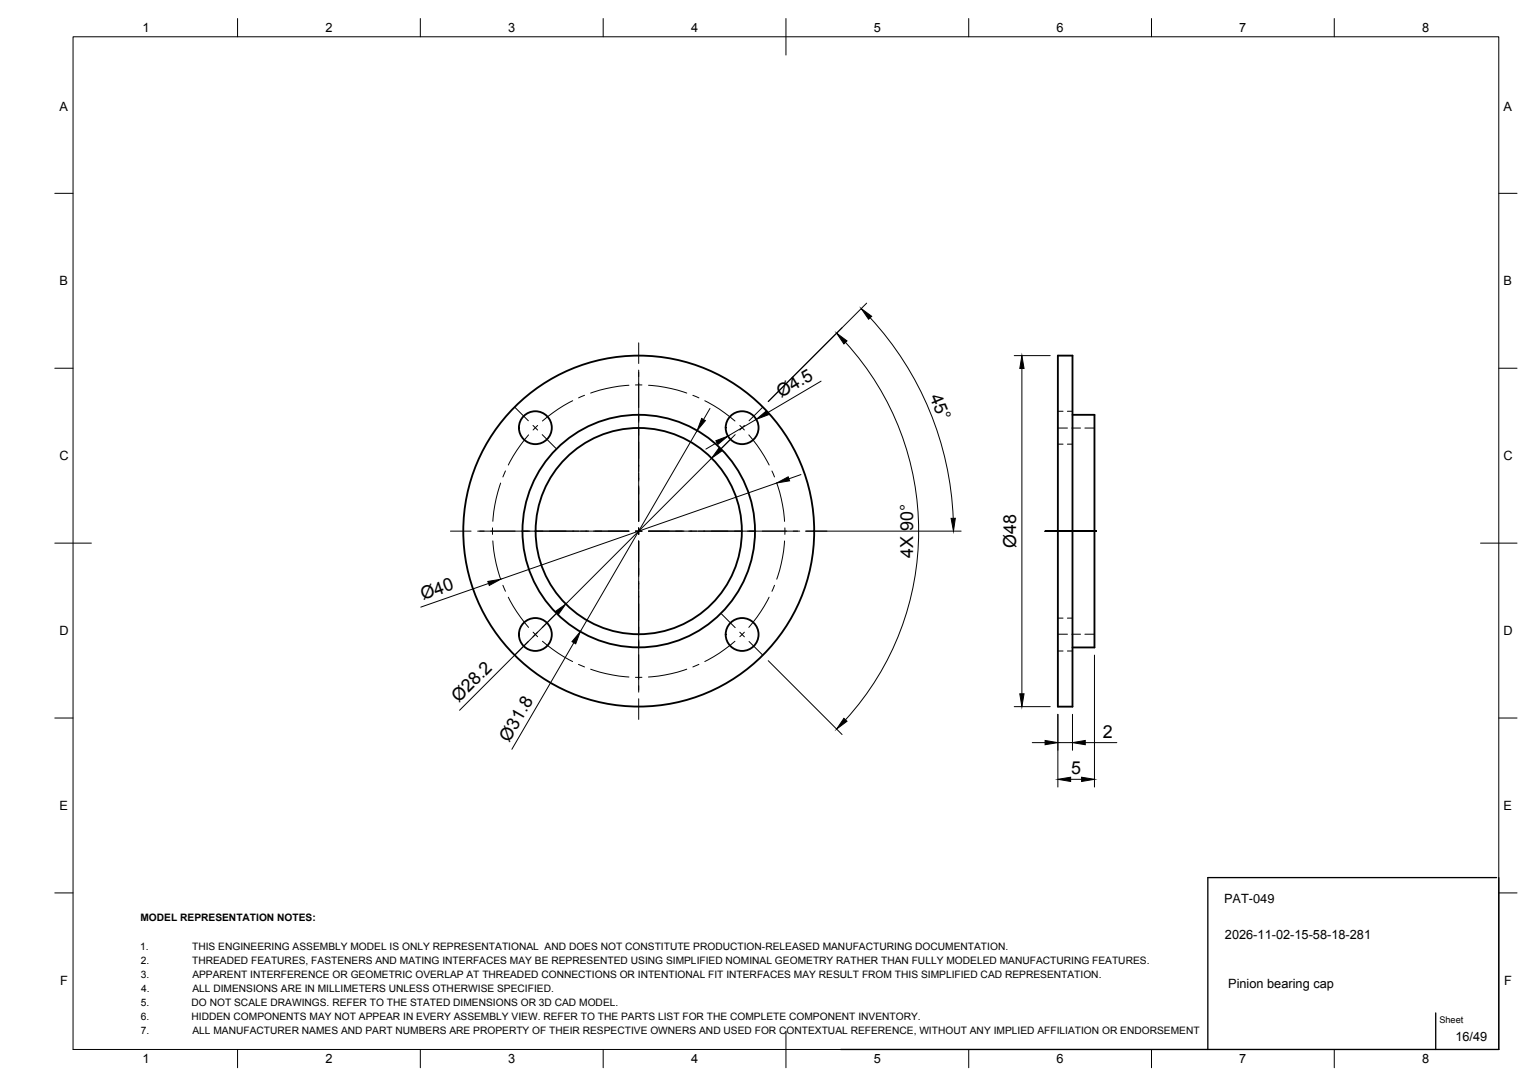
ISO-10303-21;
HEADER;
/* Generated by software containing ST-Developer
 * from STEP Tools, Inc. (www.steptools.com) 
 */

FILE_DESCRIPTION(
/* description */ ('Hand drill press frame (manual)'),
/* implementation_level */ '2;1');

FILE_NAME(
/* name */ 'Pinion bearing cap.step',
/* time_stamp */ '2026-10-28T03:25:28-07:00',
/* author */ (''),
/* organization */ (''),
/* preprocessor_version */ 'ST-DEVELOPER v20.2',
/* originating_system */ 'Autodesk Translation Framework v15.17.0.0',
/* authorisation */ '');

FILE_SCHEMA (('AUTOMOTIVE_DESIGN { 1 0 10303 214 3 1 1 }'));
ENDSEC;

DATA;
#10=MECHANICAL_DESIGN_GEOMETRIC_PRESENTATION_REPRESENTATION('',(#630),#33299);
#540=SHAPE_REPRESENTATION_RELATIONSHIP('SRR','None',#33499,#585);
#585=ADVANCED_BREP_SHAPE_REPRESENTATION('',(#682),#33261);
#630=STYLED_ITEM('',(#33814),#682);
#682=MANIFOLD_SOLID_BREP('Body1',#12648);
#778=FACE_BOUND('',#2248,.T.);
#779=FACE_BOUND('',#2252,.T.);
#780=FACE_BOUND('',#2253,.T.);
#781=FACE_BOUND('',#2254,.T.);
#782=FACE_BOUND('',#2255,.T.);
#783=FACE_BOUND('',#2256,.T.);
#784=FACE_BOUND('',#2258,.T.);
#785=FACE_BOUND('',#2259,.T.);
#786=FACE_BOUND('',#2260,.T.);
#787=FACE_BOUND('',#2261,.T.);
#788=FACE_BOUND('',#2262,.T.);
#993=PLANE('',#13479);
#994=PLANE('',#13486);
#995=PLANE('',#13487);
#1495=FACE_OUTER_BOUND('',#2242,.T.);
#1496=FACE_OUTER_BOUND('',#2243,.T.);
#1497=FACE_OUTER_BOUND('',#2244,.T.);
#1498=FACE_OUTER_BOUND('',#2245,.T.);
#1499=FACE_OUTER_BOUND('',#2246,.T.);
#1500=FACE_OUTER_BOUND('',#2247,.T.);
#1501=FACE_OUTER_BOUND('',#2249,.T.);
#1502=FACE_OUTER_BOUND('',#2250,.T.);
#1503=FACE_OUTER_BOUND('',#2251,.T.);
#1504=FACE_OUTER_BOUND('',#2257,.T.);
#2242=EDGE_LOOP('',(#9179,#9180,#9181,#9182));
#2243=EDGE_LOOP('',(#9183,#9184,#9185,#9186));
#2244=EDGE_LOOP('',(#9187,#9188,#9189,#9190));
#2245=EDGE_LOOP('',(#9191,#9192,#9193,#9194));
#2246=EDGE_LOOP('',(#9195,#9196,#9197,#9198));
#2247=EDGE_LOOP('',(#9199));
#2248=EDGE_LOOP('',(#9200));
#2249=EDGE_LOOP('',(#9201,#9202,#9203,#9204));
#2250=EDGE_LOOP('',(#9205,#9206,#9207,#9208));
#2251=EDGE_LOOP('',(#9209));
#2252=EDGE_LOOP('',(#9210));
#2253=EDGE_LOOP('',(#9211));
#2254=EDGE_LOOP('',(#9212));
#2255=EDGE_LOOP('',(#9213));
#2256=EDGE_LOOP('',(#9214));
#2257=EDGE_LOOP('',(#9215));
#2258=EDGE_LOOP('',(#9216));
#2259=EDGE_LOOP('',(#9217));
#2260=EDGE_LOOP('',(#9218));
#2261=EDGE_LOOP('',(#9219));
#2262=EDGE_LOOP('',(#9220));
#3142=LINE('',#18879,#4307);
#3143=LINE('',#18885,#4308);
#3144=LINE('',#18891,#4309);
#3145=LINE('',#18897,#4310);
#3146=LINE('',#18903,#4311);
#3147=LINE('',#18910,#4312);
#3148=LINE('',#18916,#4313);
#4307=VECTOR('',#15181,0.225);
#4308=VECTOR('',#15188,0.225);
#4309=VECTOR('',#15195,0.225);
#4310=VECTOR('',#15202,0.225);
#4311=VECTOR('',#15209,1.59);
#4312=VECTOR('',#15218,1.41);
#4313=VECTOR('',#15225,2.4);
#5320=CIRCLE('',#13465,0.225);
#5321=CIRCLE('',#13466,0.225);
#5322=CIRCLE('',#13468,0.225);
#5323=CIRCLE('',#13469,0.225);
#5324=CIRCLE('',#13471,0.225);
#5325=CIRCLE('',#13472,0.225);
#5326=CIRCLE('',#13474,0.225);
#5327=CIRCLE('',#13475,0.225);
#5328=CIRCLE('',#13477,1.59);
#5329=CIRCLE('',#13478,1.59);
#5330=CIRCLE('',#13480,1.41);
#5331=CIRCLE('',#13482,1.41);
#5332=CIRCLE('',#13484,2.4);
#5333=CIRCLE('',#13485,2.4);
#5866=VERTEX_POINT('',#18876);
#5867=VERTEX_POINT('',#18878);
#5868=VERTEX_POINT('',#18882);
#5869=VERTEX_POINT('',#18884);
#5870=VERTEX_POINT('',#18888);
#5871=VERTEX_POINT('',#18890);
#5872=VERTEX_POINT('',#18894);
#5873=VERTEX_POINT('',#18896);
#5874=VERTEX_POINT('',#18900);
#5875=VERTEX_POINT('',#18902);
#5876=VERTEX_POINT('',#18906);
#5877=VERTEX_POINT('',#18909);
#5878=VERTEX_POINT('',#18913);
#5879=VERTEX_POINT('',#18915);
#7118=EDGE_CURVE('',#5866,#5866,#5320,.T.);
#7119=EDGE_CURVE('',#5866,#5867,#3142,.T.);
#7120=EDGE_CURVE('',#5867,#5867,#5321,.T.);
#7121=EDGE_CURVE('',#5868,#5868,#5322,.T.);
#7122=EDGE_CURVE('',#5868,#5869,#3143,.T.);
#7123=EDGE_CURVE('',#5869,#5869,#5323,.T.);
#7124=EDGE_CURVE('',#5870,#5870,#5324,.T.);
#7125=EDGE_CURVE('',#5870,#5871,#3144,.T.);
#7126=EDGE_CURVE('',#5871,#5871,#5325,.T.);
#7127=EDGE_CURVE('',#5872,#5872,#5326,.T.);
#7128=EDGE_CURVE('',#5872,#5873,#3145,.T.);
#7129=EDGE_CURVE('',#5873,#5873,#5327,.T.);
#7130=EDGE_CURVE('',#5874,#5874,#5328,.T.);
#7131=EDGE_CURVE('',#5874,#5875,#3146,.T.);
#7132=EDGE_CURVE('',#5875,#5875,#5329,.T.);
#7133=EDGE_CURVE('',#5876,#5876,#5330,.T.);
#7134=EDGE_CURVE('',#5876,#5877,#3147,.T.);
#7135=EDGE_CURVE('',#5877,#5877,#5331,.T.);
#7136=EDGE_CURVE('',#5878,#5878,#5332,.T.);
#7137=EDGE_CURVE('',#5878,#5879,#3148,.T.);
#7138=EDGE_CURVE('',#5879,#5879,#5333,.T.);
#9179=ORIENTED_EDGE('',*,*,#7118,.F.);
#9180=ORIENTED_EDGE('',*,*,#7119,.T.);
#9181=ORIENTED_EDGE('',*,*,#7120,.F.);
#9182=ORIENTED_EDGE('',*,*,#7119,.F.);
#9183=ORIENTED_EDGE('',*,*,#7121,.F.);
#9184=ORIENTED_EDGE('',*,*,#7122,.T.);
#9185=ORIENTED_EDGE('',*,*,#7123,.F.);
#9186=ORIENTED_EDGE('',*,*,#7122,.F.);
#9187=ORIENTED_EDGE('',*,*,#7124,.F.);
#9188=ORIENTED_EDGE('',*,*,#7125,.T.);
#9189=ORIENTED_EDGE('',*,*,#7126,.F.);
#9190=ORIENTED_EDGE('',*,*,#7125,.F.);
#9191=ORIENTED_EDGE('',*,*,#7127,.F.);
#9192=ORIENTED_EDGE('',*,*,#7128,.T.);
#9193=ORIENTED_EDGE('',*,*,#7129,.F.);
#9194=ORIENTED_EDGE('',*,*,#7128,.F.);
#9195=ORIENTED_EDGE('',*,*,#7130,.F.);
#9196=ORIENTED_EDGE('',*,*,#7131,.T.);
#9197=ORIENTED_EDGE('',*,*,#7132,.F.);
#9198=ORIENTED_EDGE('',*,*,#7131,.F.);
#9199=ORIENTED_EDGE('',*,*,#7130,.T.);
#9200=ORIENTED_EDGE('',*,*,#7133,.T.);
#9201=ORIENTED_EDGE('',*,*,#7133,.F.);
#9202=ORIENTED_EDGE('',*,*,#7134,.T.);
#9203=ORIENTED_EDGE('',*,*,#7135,.T.);
#9204=ORIENTED_EDGE('',*,*,#7134,.F.);
#9205=ORIENTED_EDGE('',*,*,#7136,.F.);
#9206=ORIENTED_EDGE('',*,*,#7137,.T.);
#9207=ORIENTED_EDGE('',*,*,#7138,.T.);
#9208=ORIENTED_EDGE('',*,*,#7137,.F.);
#9209=ORIENTED_EDGE('',*,*,#7136,.T.);
#9210=ORIENTED_EDGE('',*,*,#7132,.T.);
#9211=ORIENTED_EDGE('',*,*,#7129,.T.);
#9212=ORIENTED_EDGE('',*,*,#7126,.T.);
#9213=ORIENTED_EDGE('',*,*,#7123,.T.);
#9214=ORIENTED_EDGE('',*,*,#7120,.T.);
#9215=ORIENTED_EDGE('',*,*,#7138,.F.);
#9216=ORIENTED_EDGE('',*,*,#7135,.F.);
#9217=ORIENTED_EDGE('',*,*,#7127,.T.);
#9218=ORIENTED_EDGE('',*,*,#7124,.T.);
#9219=ORIENTED_EDGE('',*,*,#7121,.T.);
#9220=ORIENTED_EDGE('',*,*,#7118,.T.);
#11835=CYLINDRICAL_SURFACE('',#13464,0.225);
#11836=CYLINDRICAL_SURFACE('',#13467,0.225);
#11837=CYLINDRICAL_SURFACE('',#13470,0.225);
#11838=CYLINDRICAL_SURFACE('',#13473,0.225);
#11839=CYLINDRICAL_SURFACE('',#13476,1.59);
#11840=CYLINDRICAL_SURFACE('',#13481,1.41);
#11841=CYLINDRICAL_SURFACE('',#13483,2.4);
#12104=ADVANCED_FACE('',(#1495),#11835,.F.);
#12105=ADVANCED_FACE('',(#1496),#11836,.F.);
#12106=ADVANCED_FACE('',(#1497),#11837,.F.);
#12107=ADVANCED_FACE('',(#1498),#11838,.F.);
#12108=ADVANCED_FACE('',(#1499),#11839,.T.);
#12109=ADVANCED_FACE('',(#1500,#778),#993,.T.);
#12110=ADVANCED_FACE('',(#1501),#11840,.F.);
#12111=ADVANCED_FACE('',(#1502),#11841,.T.);
#12112=ADVANCED_FACE('',(#1503,#779,#780,#781,#782,#783),#994,.T.);
#12113=ADVANCED_FACE('',(#1504,#784,#785,#786,#787,#788),#995,.F.);
#12648=CLOSED_SHELL('',(#12104,#12105,#12106,#12107,#12108,#12109,#12110,
#12111,#12112,#12113));
#13463=AXIS2_PLACEMENT_3D('',#18874,#15175,#15176);
#13464=AXIS2_PLACEMENT_3D('',#18875,#15177,#15178);
#13465=AXIS2_PLACEMENT_3D('',#18877,#15179,#15180);
#13466=AXIS2_PLACEMENT_3D('',#18880,#15182,#15183);
#13467=AXIS2_PLACEMENT_3D('',#18881,#15184,#15185);
#13468=AXIS2_PLACEMENT_3D('',#18883,#15186,#15187);
#13469=AXIS2_PLACEMENT_3D('',#18886,#15189,#15190);
#13470=AXIS2_PLACEMENT_3D('',#18887,#15191,#15192);
#13471=AXIS2_PLACEMENT_3D('',#18889,#15193,#15194);
#13472=AXIS2_PLACEMENT_3D('',#18892,#15196,#15197);
#13473=AXIS2_PLACEMENT_3D('',#18893,#15198,#15199);
#13474=AXIS2_PLACEMENT_3D('',#18895,#15200,#15201);
#13475=AXIS2_PLACEMENT_3D('',#18898,#15203,#15204);
#13476=AXIS2_PLACEMENT_3D('',#18899,#15205,#15206);
#13477=AXIS2_PLACEMENT_3D('',#18901,#15207,#15208);
#13478=AXIS2_PLACEMENT_3D('',#18904,#15210,#15211);
#13479=AXIS2_PLACEMENT_3D('',#18905,#15212,#15213);
#13480=AXIS2_PLACEMENT_3D('',#18907,#15214,#15215);
#13481=AXIS2_PLACEMENT_3D('',#18908,#15216,#15217);
#13482=AXIS2_PLACEMENT_3D('',#18911,#15219,#15220);
#13483=AXIS2_PLACEMENT_3D('',#18912,#15221,#15222);
#13484=AXIS2_PLACEMENT_3D('',#18914,#15223,#15224);
#13485=AXIS2_PLACEMENT_3D('',#18917,#15226,#15227);
#13486=AXIS2_PLACEMENT_3D('',#18918,#15228,#15229);
#13487=AXIS2_PLACEMENT_3D('',#18919,#15230,#15231);
#15175=DIRECTION('axis',(0.,0.,1.));
#15176=DIRECTION('refdir',(1.,0.,0.));
#15177=DIRECTION('center_axis',(0.,1.,0.));
#15178=DIRECTION('ref_axis',(1.,0.,0.));
#15179=DIRECTION('center_axis',(0.,1.,0.));
#15180=DIRECTION('ref_axis',(1.,0.,0.));
#15181=DIRECTION('',(0.,1.,0.));
#15182=DIRECTION('center_axis',(0.,-1.,0.));
#15183=DIRECTION('ref_axis',(1.,0.,0.));
#15184=DIRECTION('center_axis',(0.,1.,0.));
#15185=DIRECTION('ref_axis',(1.,0.,0.));
#15186=DIRECTION('center_axis',(0.,1.,0.));
#15187=DIRECTION('ref_axis',(1.,0.,0.));
#15188=DIRECTION('',(0.,1.,0.));
#15189=DIRECTION('center_axis',(0.,-1.,0.));
#15190=DIRECTION('ref_axis',(1.,0.,0.));
#15191=DIRECTION('center_axis',(0.,1.,0.));
#15192=DIRECTION('ref_axis',(1.,0.,0.));
#15193=DIRECTION('center_axis',(0.,1.,0.));
#15194=DIRECTION('ref_axis',(1.,0.,0.));
#15195=DIRECTION('',(0.,1.,0.));
#15196=DIRECTION('center_axis',(0.,-1.,0.));
#15197=DIRECTION('ref_axis',(1.,0.,0.));
#15198=DIRECTION('center_axis',(0.,1.,0.));
#15199=DIRECTION('ref_axis',(1.,0.,0.));
#15200=DIRECTION('center_axis',(0.,1.,0.));
#15201=DIRECTION('ref_axis',(1.,0.,0.));
#15202=DIRECTION('',(0.,1.,0.));
#15203=DIRECTION('center_axis',(0.,-1.,0.));
#15204=DIRECTION('ref_axis',(1.,0.,0.));
#15205=DIRECTION('center_axis',(0.,1.,0.));
#15206=DIRECTION('ref_axis',(1.,0.,0.));
#15207=DIRECTION('center_axis',(0.,1.,0.));
#15208=DIRECTION('ref_axis',(1.,0.,0.));
#15209=DIRECTION('',(0.,-1.,0.));
#15210=DIRECTION('center_axis',(0.,-1.,0.));
#15211=DIRECTION('ref_axis',(1.,0.,0.));
#15212=DIRECTION('center_axis',(0.,1.,0.));
#15213=DIRECTION('ref_axis',(1.,0.,0.));
#15214=DIRECTION('center_axis',(0.,-1.,0.));
#15215=DIRECTION('ref_axis',(1.,0.,0.));
#15216=DIRECTION('center_axis',(0.,1.,0.));
#15217=DIRECTION('ref_axis',(1.,0.,0.));
#15218=DIRECTION('',(0.,-1.,0.));
#15219=DIRECTION('center_axis',(0.,-1.,0.));
#15220=DIRECTION('ref_axis',(1.,0.,0.));
#15221=DIRECTION('center_axis',(0.,1.,0.));
#15222=DIRECTION('ref_axis',(1.,0.,0.));
#15223=DIRECTION('center_axis',(0.,1.,0.));
#15224=DIRECTION('ref_axis',(1.,0.,0.));
#15225=DIRECTION('',(0.,-1.,0.));
#15226=DIRECTION('center_axis',(0.,1.,0.));
#15227=DIRECTION('ref_axis',(1.,0.,0.));
#15228=DIRECTION('center_axis',(0.,1.,0.));
#15229=DIRECTION('ref_axis',(1.,0.,0.));
#15230=DIRECTION('center_axis',(0.,1.,0.));
#15231=DIRECTION('ref_axis',(1.,0.,0.));
#18874=CARTESIAN_POINT('',(0.,0.,0.));
#18875=CARTESIAN_POINT('Origin',(-4.66421356237309,-4.1,18.5857864376269));
#18876=CARTESIAN_POINT('',(-4.88921356237309,-4.,18.5857864376269));
#18877=CARTESIAN_POINT('Origin',(-4.66421356237309,-4.,18.5857864376269));
#18878=CARTESIAN_POINT('',(-4.88921356237309,-3.8,18.5857864376269));
#18879=CARTESIAN_POINT('',(-4.88921356237309,-4.1,18.5857864376269));
#18880=CARTESIAN_POINT('Origin',(-4.66421356237309,-3.8,18.5857864376269));
#18881=CARTESIAN_POINT('Origin',(-4.66421356237309,-4.1,21.4142135623731));
#18882=CARTESIAN_POINT('',(-4.88921356237309,-4.,21.4142135623731));
#18883=CARTESIAN_POINT('Origin',(-4.66421356237309,-4.,21.4142135623731));
#18884=CARTESIAN_POINT('',(-4.88921356237309,-3.8,21.4142135623731));
#18885=CARTESIAN_POINT('',(-4.88921356237309,-4.1,21.4142135623731));
#18886=CARTESIAN_POINT('Origin',(-4.66421356237309,-3.8,21.4142135623731));
#18887=CARTESIAN_POINT('Origin',(-1.8357864376269,-4.1,21.4142135623731));
#18888=CARTESIAN_POINT('',(-2.0607864376269,-4.,21.4142135623731));
#18889=CARTESIAN_POINT('Origin',(-1.8357864376269,-4.,21.4142135623731));
#18890=CARTESIAN_POINT('',(-2.0607864376269,-3.8,21.4142135623731));
#18891=CARTESIAN_POINT('',(-2.0607864376269,-4.1,21.4142135623731));
#18892=CARTESIAN_POINT('Origin',(-1.8357864376269,-3.8,21.4142135623731));
#18893=CARTESIAN_POINT('Origin',(-1.83578643762691,-4.1,18.5857864376269));
#18894=CARTESIAN_POINT('',(-2.06078643762691,-4.,18.5857864376269));
#18895=CARTESIAN_POINT('Origin',(-1.83578643762691,-4.,18.5857864376269));
#18896=CARTESIAN_POINT('',(-2.06078643762691,-3.8,18.5857864376269));
#18897=CARTESIAN_POINT('',(-2.06078643762691,-4.1,18.5857864376269));
#18898=CARTESIAN_POINT('Origin',(-1.83578643762691,-3.8,18.5857864376269));
#18899=CARTESIAN_POINT('Origin',(-3.25,-3.8,20.));
#18900=CARTESIAN_POINT('',(-4.84,-3.5,20.));
#18901=CARTESIAN_POINT('Origin',(-3.25,-3.5,20.));
#18902=CARTESIAN_POINT('',(-4.84,-3.8,20.));
#18903=CARTESIAN_POINT('',(-4.84,-3.8,20.));
#18904=CARTESIAN_POINT('Origin',(-3.25,-3.8,20.));
#18905=CARTESIAN_POINT('Origin',(-3.25,-3.5,20.));
#18906=CARTESIAN_POINT('',(-4.66,-3.5,20.));
#18907=CARTESIAN_POINT('Origin',(-3.25,-3.5,20.));
#18908=CARTESIAN_POINT('Origin',(-3.25,-4.,20.));
#18909=CARTESIAN_POINT('',(-4.66,-4.,20.));
#18910=CARTESIAN_POINT('',(-4.66,-4.,20.));
#18911=CARTESIAN_POINT('Origin',(-3.25,-4.,20.));
#18912=CARTESIAN_POINT('Origin',(-3.25,-4.,20.));
#18913=CARTESIAN_POINT('',(-5.65,-3.8,20.));
#18914=CARTESIAN_POINT('Origin',(-3.25,-3.8,20.));
#18915=CARTESIAN_POINT('',(-5.65,-4.,20.));
#18916=CARTESIAN_POINT('',(-5.65,-4.,20.));
#18917=CARTESIAN_POINT('Origin',(-3.25,-4.,20.));
#18918=CARTESIAN_POINT('Origin',(-3.25,-3.8,20.));
#18919=CARTESIAN_POINT('Origin',(-3.25,-4.,20.));
#33209=UNCERTAINTY_MEASURE_WITH_UNIT(LENGTH_MEASURE(0.001),#33300,
'DISTANCE_ACCURACY_VALUE',
'Maximum model space distance between geometric entities at asserted c
onnectivities');
#33247=UNCERTAINTY_MEASURE_WITH_UNIT(LENGTH_MEASURE(0.001),#33300,
'DISTANCE_ACCURACY_VALUE',
'Maximum model space distance between geometric entities at asserted c
onnectivities');
#33261=(
GEOMETRIC_REPRESENTATION_CONTEXT(3)
GLOBAL_UNCERTAINTY_ASSIGNED_CONTEXT((#33209))
GLOBAL_UNIT_ASSIGNED_CONTEXT((#33300,#33302,#33303))
REPRESENTATION_CONTEXT('','3D')
);
#33299=(
GEOMETRIC_REPRESENTATION_CONTEXT(3)
GLOBAL_UNCERTAINTY_ASSIGNED_CONTEXT((#33247))
GLOBAL_UNIT_ASSIGNED_CONTEXT((#33300,#33302,#33303))
REPRESENTATION_CONTEXT('','3D')
);
#33300=(
LENGTH_UNIT()
NAMED_UNIT(*)
SI_UNIT(.CENTI.,.METRE.)
);
#33302=(
NAMED_UNIT(*)
PLANE_ANGLE_UNIT()
SI_UNIT($,.RADIAN.)
);
#33303=(
NAMED_UNIT(*)
SI_UNIT($,.STERADIAN.)
SOLID_ANGLE_UNIT()
);
#33317=SHAPE_DEFINITION_REPRESENTATION(#33368,#33499);
#33368=PRODUCT_DEFINITION_SHAPE('',$,#33551);
#33499=SHAPE_REPRESENTATION('',(#13463),#33261);
#33537=PRODUCT_DEFINITION_CONTEXT('part definition',#33692,'design');
#33551=PRODUCT_DEFINITION('Pinion bearing cap','Pinion bearing cap',#33602,
#33537);
#33602=PRODUCT_DEFINITION_FORMATION('',$,#33707);
#33692=APPLICATION_CONTEXT(
'Core Data for Automotive Mechanical Design Process');
#33693=PRODUCT_CONTEXT('part definition',#33692,'mechanical');
#33707=PRODUCT('Pinion bearing cap','Pinion bearing cap',
'Pinion bearing cap',(#33693));
#33808=COLOUR_RGB('Grey',0.48,0.52,0.57);
#33809=FILL_AREA_STYLE_COLOUR('',#33808);
#33810=FILL_AREA_STYLE('',(#33809));
#33811=SURFACE_STYLE_FILL_AREA(#33810);
#33812=SURFACE_SIDE_STYLE('',(#33811));
#33813=SURFACE_STYLE_USAGE(.BOTH.,#33812);
#33814=PRESENTATION_STYLE_ASSIGNMENT((#33813));
ENDSEC;
END-ISO-10303-21;
